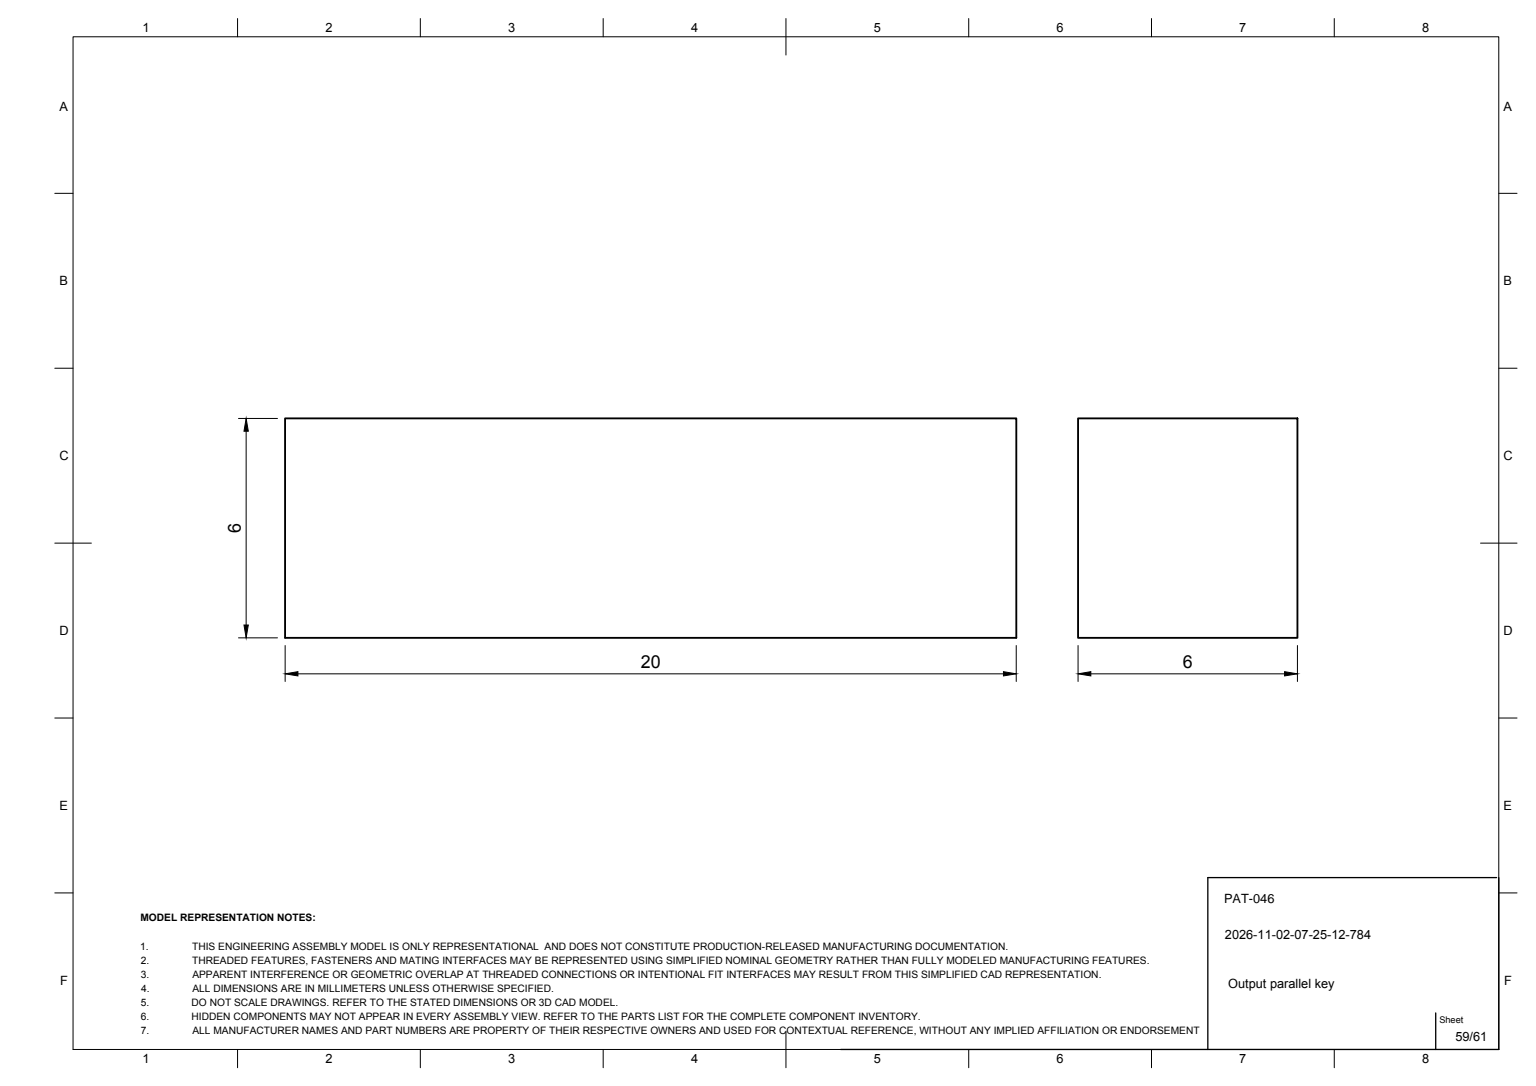
ISO-10303-21;
HEADER;
/* Generated by software containing ST-Developer
 * from STEP Tools, Inc. (www.steptools.com) 
 */

FILE_DESCRIPTION(
/* description */ ('Gear mesh backlash fixture'),
/* implementation_level */ '2;1');

FILE_NAME(
/* name */ 'Output parallel key.step',
/* time_stamp */ '2026-10-28T03:26:00-07:00',
/* author */ (''),
/* organization */ (''),
/* preprocessor_version */ 'ST-DEVELOPER v20.2',
/* originating_system */ 'Autodesk Translation Framework v15.17.0.0',
/* authorisation */ '');

FILE_SCHEMA (('AUTOMOTIVE_DESIGN { 1 0 10303 214 3 1 1 }'));
ENDSEC;

DATA;
#10=MECHANICAL_DESIGN_GEOMETRIC_PRESENTATION_REPRESENTATION('',(#1076),#57900);
#961=SHAPE_REPRESENTATION_RELATIONSHIP('SRR','None',#58162,#1011);
#1011=ADVANCED_BREP_SHAPE_REPRESENTATION('',(#1139),#57895);
#1076=STYLED_ITEM('',(#58465),#1139);
#1139=MANIFOLD_SOLID_BREP('Body1',#13638);
#1620=PLANE('',#15276);
#1621=PLANE('',#15277);
#1622=PLANE('',#15278);
#1623=PLANE('',#15279);
#1624=PLANE('',#15280);
#1625=PLANE('',#15281);
#2254=FACE_OUTER_BOUND('',#3199,.T.);
#2255=FACE_OUTER_BOUND('',#3200,.T.);
#2256=FACE_OUTER_BOUND('',#3201,.T.);
#2257=FACE_OUTER_BOUND('',#3202,.T.);
#2258=FACE_OUTER_BOUND('',#3203,.T.);
#2259=FACE_OUTER_BOUND('',#3204,.T.);
#3199=EDGE_LOOP('',(#11453,#11454,#11455,#11456));
#3200=EDGE_LOOP('',(#11457,#11458,#11459,#11460));
#3201=EDGE_LOOP('',(#11461,#11462,#11463,#11464));
#3202=EDGE_LOOP('',(#11465,#11466,#11467,#11468));
#3203=EDGE_LOOP('',(#11469,#11470,#11471,#11472));
#3204=EDGE_LOOP('',(#11473,#11474,#11475,#11476));
#4072=LINE('',#34000,#4961);
#4073=LINE('',#34002,#4962);
#4074=LINE('',#34004,#4963);
#4075=LINE('',#34005,#4964);
#4076=LINE('',#34008,#4965);
#4077=LINE('',#34010,#4966);
#4078=LINE('',#34011,#4967);
#4079=LINE('',#34014,#4968);
#4080=LINE('',#34016,#4969);
#4081=LINE('',#34017,#4970);
#4082=LINE('',#34019,#4971);
#4083=LINE('',#34020,#4972);
#4961=VECTOR('',#18403,1.);
#4962=VECTOR('',#18404,1.);
#4963=VECTOR('',#18405,1.);
#4964=VECTOR('',#18406,1.);
#4965=VECTOR('',#18409,1.);
#4966=VECTOR('',#18410,1.);
#4967=VECTOR('',#18411,1.);
#4968=VECTOR('',#18414,1.);
#4969=VECTOR('',#18415,1.);
#4970=VECTOR('',#18416,1.);
#4971=VECTOR('',#18419,1.);
#4972=VECTOR('',#18420,1.);
#6650=VERTEX_POINT('',#33998);
#6651=VERTEX_POINT('',#33999);
#6652=VERTEX_POINT('',#34001);
#6653=VERTEX_POINT('',#34003);
#6654=VERTEX_POINT('',#34007);
#6655=VERTEX_POINT('',#34009);
#6656=VERTEX_POINT('',#34013);
#6657=VERTEX_POINT('',#34015);
#8313=EDGE_CURVE('',#6650,#6651,#4072,.T.);
#8314=EDGE_CURVE('',#6650,#6652,#4073,.T.);
#8315=EDGE_CURVE('',#6653,#6652,#4074,.T.);
#8316=EDGE_CURVE('',#6651,#6653,#4075,.T.);
#8317=EDGE_CURVE('',#6651,#6654,#4076,.T.);
#8318=EDGE_CURVE('',#6655,#6653,#4077,.T.);
#8319=EDGE_CURVE('',#6654,#6655,#4078,.T.);
#8320=EDGE_CURVE('',#6654,#6656,#4079,.T.);
#8321=EDGE_CURVE('',#6657,#6655,#4080,.T.);
#8322=EDGE_CURVE('',#6656,#6657,#4081,.T.);
#8323=EDGE_CURVE('',#6656,#6650,#4082,.T.);
#8324=EDGE_CURVE('',#6652,#6657,#4083,.T.);
#11453=ORIENTED_EDGE('',*,*,#8313,.F.);
#11454=ORIENTED_EDGE('',*,*,#8314,.T.);
#11455=ORIENTED_EDGE('',*,*,#8315,.F.);
#11456=ORIENTED_EDGE('',*,*,#8316,.F.);
#11457=ORIENTED_EDGE('',*,*,#8317,.F.);
#11458=ORIENTED_EDGE('',*,*,#8316,.T.);
#11459=ORIENTED_EDGE('',*,*,#8318,.F.);
#11460=ORIENTED_EDGE('',*,*,#8319,.F.);
#11461=ORIENTED_EDGE('',*,*,#8320,.F.);
#11462=ORIENTED_EDGE('',*,*,#8319,.T.);
#11463=ORIENTED_EDGE('',*,*,#8321,.F.);
#11464=ORIENTED_EDGE('',*,*,#8322,.F.);
#11465=ORIENTED_EDGE('',*,*,#8323,.F.);
#11466=ORIENTED_EDGE('',*,*,#8322,.T.);
#11467=ORIENTED_EDGE('',*,*,#8324,.F.);
#11468=ORIENTED_EDGE('',*,*,#8314,.F.);
#11469=ORIENTED_EDGE('',*,*,#8324,.T.);
#11470=ORIENTED_EDGE('',*,*,#8321,.T.);
#11471=ORIENTED_EDGE('',*,*,#8318,.T.);
#11472=ORIENTED_EDGE('',*,*,#8315,.T.);
#11473=ORIENTED_EDGE('',*,*,#8323,.T.);
#11474=ORIENTED_EDGE('',*,*,#8313,.T.);
#11475=ORIENTED_EDGE('',*,*,#8317,.T.);
#11476=ORIENTED_EDGE('',*,*,#8320,.T.);
#13371=ADVANCED_FACE('',(#2254),#1620,.T.);
#13372=ADVANCED_FACE('',(#2255),#1621,.T.);
#13373=ADVANCED_FACE('',(#2256),#1622,.T.);
#13374=ADVANCED_FACE('',(#2257),#1623,.T.);
#13375=ADVANCED_FACE('',(#2258),#1624,.T.);
#13376=ADVANCED_FACE('',(#2259),#1625,.F.);
#13638=CLOSED_SHELL('',(#13371,#13372,#13373,#13374,#13375,#13376));
#15275=AXIS2_PLACEMENT_3D('',#33996,#18399,#18400);
#15276=AXIS2_PLACEMENT_3D('',#33997,#18401,#18402);
#15277=AXIS2_PLACEMENT_3D('',#34006,#18407,#18408);
#15278=AXIS2_PLACEMENT_3D('',#34012,#18412,#18413);
#15279=AXIS2_PLACEMENT_3D('',#34018,#18417,#18418);
#15280=AXIS2_PLACEMENT_3D('',#34021,#18421,#18422);
#15281=AXIS2_PLACEMENT_3D('',#34022,#18423,#18424);
#18399=DIRECTION('axis',(0.,0.,1.));
#18400=DIRECTION('refdir',(1.,0.,0.));
#18401=DIRECTION('center_axis',(0.0784590957278448,-0.996917333733128,0.));
#18402=DIRECTION('ref_axis',(0.996917333733128,0.0784590957278448,0.));
#18403=DIRECTION('',(-0.996917333733128,-0.0784590957278448,0.));
#18404=DIRECTION('',(0.,0.,1.));
#18405=DIRECTION('',(0.996917333733128,0.0784590957278448,0.));
#18406=DIRECTION('',(0.,0.,1.));
#18407=DIRECTION('center_axis',(-0.996917333733128,-0.078459095727846,0.));
#18408=DIRECTION('ref_axis',(0.078459095727846,-0.996917333733128,0.));
#18409=DIRECTION('',(-0.078459095727846,0.996917333733128,0.));
#18410=DIRECTION('',(0.078459095727846,-0.996917333733128,0.));
#18411=DIRECTION('',(0.,0.,1.));
#18412=DIRECTION('center_axis',(-0.078459095727845,0.996917333733128,0.));
#18413=DIRECTION('ref_axis',(-0.996917333733128,-0.078459095727845,0.));
#18414=DIRECTION('',(0.996917333733128,0.078459095727845,0.));
#18415=DIRECTION('',(-0.996917333733128,-0.078459095727845,0.));
#18416=DIRECTION('',(0.,0.,1.));
#18417=DIRECTION('center_axis',(0.996917333733128,0.078459095727846,0.));
#18418=DIRECTION('ref_axis',(-0.078459095727846,0.996917333733128,0.));
#18419=DIRECTION('',(0.078459095727846,-0.996917333733128,0.));
#18420=DIRECTION('',(-0.078459095727846,0.996917333733128,0.));
#18421=DIRECTION('center_axis',(0.,0.,1.));
#18422=DIRECTION('ref_axis',(1.,0.,0.));
#18423=DIRECTION('center_axis',(0.,0.,1.));
#18424=DIRECTION('ref_axis',(1.,0.,0.));
#33996=CARTESIAN_POINT('',(0.,0.,0.));
#33997=CARTESIAN_POINT('Origin',(5.64992638765696,0.62445853820818,11.5));
#33998=CARTESIAN_POINT('',(6.24807678789684,0.671533995644887,11.5));
#33999=CARTESIAN_POINT('',(5.64992638765696,0.62445853820818,11.5));
#34000=CARTESIAN_POINT('',(6.24807678789684,0.671533995644887,11.5));
#34001=CARTESIAN_POINT('',(6.24807678789684,0.671533995644887,13.5));
#34002=CARTESIAN_POINT('',(6.24807678789684,0.671533995644887,11.5));
#34003=CARTESIAN_POINT('',(5.64992638765696,0.62445853820818,13.5));
#34004=CARTESIAN_POINT('',(6.24807678789684,0.671533995644887,13.5));
#34005=CARTESIAN_POINT('',(5.64992638765696,0.62445853820818,11.5));
#34006=CARTESIAN_POINT('Origin',(5.60285093022026,1.22260893844806,11.5));
#34007=CARTESIAN_POINT('',(5.60285093022026,1.22260893844806,11.5));
#34008=CARTESIAN_POINT('',(5.64992638765696,0.62445853820818,11.5));
#34009=CARTESIAN_POINT('',(5.60285093022026,1.22260893844806,13.5));
#34010=CARTESIAN_POINT('',(5.64992638765696,0.62445853820818,13.5));
#34011=CARTESIAN_POINT('',(5.60285093022026,1.22260893844806,11.5));
#34012=CARTESIAN_POINT('Origin',(6.20100133046013,1.26968439588476,11.5));
#34013=CARTESIAN_POINT('',(6.20100133046013,1.26968439588476,11.5));
#34014=CARTESIAN_POINT('',(5.60285093022026,1.22260893844806,11.5));
#34015=CARTESIAN_POINT('',(6.20100133046013,1.26968439588476,13.5));
#34016=CARTESIAN_POINT('',(5.60285093022026,1.22260893844806,13.5));
#34017=CARTESIAN_POINT('',(6.20100133046013,1.26968439588476,11.5));
#34018=CARTESIAN_POINT('Origin',(6.24807678789684,0.671533995644887,11.5));
#34019=CARTESIAN_POINT('',(6.20100133046013,1.26968439588476,11.5));
#34020=CARTESIAN_POINT('',(6.20100133046013,1.26968439588476,13.5));
#34021=CARTESIAN_POINT('Origin',(5.92546385905855,0.947071467046472,13.5));
#34022=CARTESIAN_POINT('Origin',(5.92546385905855,0.947071467046472,11.5));
#57836=UNCERTAINTY_MEASURE_WITH_UNIT(LENGTH_MEASURE(0.001),#57901,
'DISTANCE_ACCURACY_VALUE',
'Maximum model space distance between geometric entities at asserted c
onnectivities');
#57841=UNCERTAINTY_MEASURE_WITH_UNIT(LENGTH_MEASURE(0.001),#57901,
'DISTANCE_ACCURACY_VALUE',
'Maximum model space distance between geometric entities at asserted c
onnectivities');
#57895=(
GEOMETRIC_REPRESENTATION_CONTEXT(3)
GLOBAL_UNCERTAINTY_ASSIGNED_CONTEXT((#57836))
GLOBAL_UNIT_ASSIGNED_CONTEXT((#57901,#57903,#57904))
REPRESENTATION_CONTEXT('','3D')
);
#57900=(
GEOMETRIC_REPRESENTATION_CONTEXT(3)
GLOBAL_UNCERTAINTY_ASSIGNED_CONTEXT((#57841))
GLOBAL_UNIT_ASSIGNED_CONTEXT((#57901,#57903,#57904))
REPRESENTATION_CONTEXT('','3D')
);
#57901=(
LENGTH_UNIT()
NAMED_UNIT(*)
SI_UNIT(.CENTI.,.METRE.)
);
#57903=(
NAMED_UNIT(*)
PLANE_ANGLE_UNIT()
SI_UNIT($,.RADIAN.)
);
#57904=(
NAMED_UNIT(*)
SI_UNIT($,.STERADIAN.)
SOLID_ANGLE_UNIT()
);
#57958=SHAPE_DEFINITION_REPRESENTATION(#58029,#58162);
#58029=PRODUCT_DEFINITION_SHAPE('',$,#58221);
#58162=SHAPE_REPRESENTATION('',(#15275),#57895);
#58167=PRODUCT_DEFINITION_CONTEXT('part definition',#58343,'design');
#58221=PRODUCT_DEFINITION('Output parallel key','Output parallel key',#58279,
#58167);
#58279=PRODUCT_DEFINITION_FORMATION('',$,#58398);
#58343=APPLICATION_CONTEXT(
'Core Data for Automotive Mechanical Design Process');
#58344=PRODUCT_CONTEXT('part definition',#58343,'mechanical');
#58398=PRODUCT('Output parallel key','Output parallel key',
'Output parallel key',(#58344));
#58459=COLOUR_RGB('Grey',0.48,0.52,0.57);
#58460=FILL_AREA_STYLE_COLOUR('',#58459);
#58461=FILL_AREA_STYLE('',(#58460));
#58462=SURFACE_STYLE_FILL_AREA(#58461);
#58463=SURFACE_SIDE_STYLE('',(#58462));
#58464=SURFACE_STYLE_USAGE(.BOTH.,#58463);
#58465=PRESENTATION_STYLE_ASSIGNMENT((#58464));
ENDSEC;
END-ISO-10303-21;
